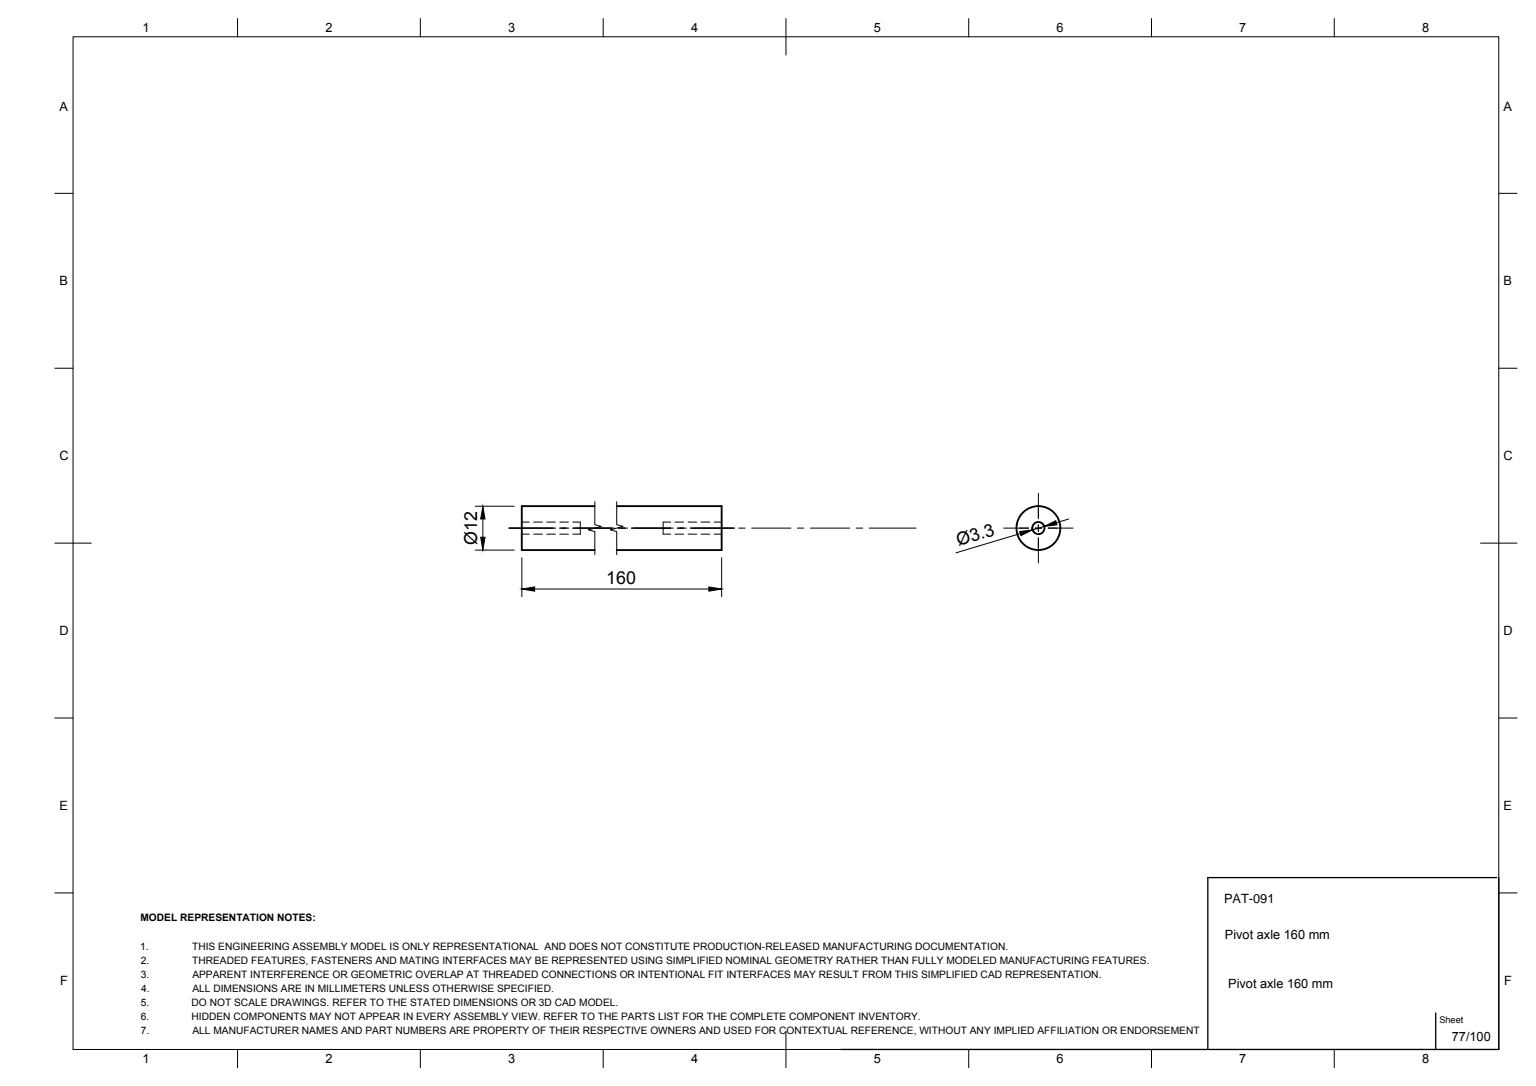
ISO-10303-21;
HEADER;
/* Generated by software containing ST-Developer
 * from STEP Tools, Inc. (www.steptools.com) 
 */

FILE_DESCRIPTION(
/* description */ ('PAT-091'),
/* implementation_level */ '2;1');

FILE_NAME(
/* name */ 'Pivot axle 160 mm.step',
/* time_stamp */ '2026-10-27T15:34:44-07:00',
/* author */ (''),
/* organization */ (''),
/* preprocessor_version */ 'ST-DEVELOPER v20.2',
/* originating_system */ 'Autodesk Translation Framework v15.17.0.0',
/* authorisation */ '');

FILE_SCHEMA (('AUTOMOTIVE_DESIGN { 1 0 10303 214 3 1 1 }'));
ENDSEC;

DATA;
#10=MECHANICAL_DESIGN_GEOMETRIC_PRESENTATION_REPRESENTATION('',(#1035),#25100);
#815=SHAPE_REPRESENTATION_RELATIONSHIP('SRR','None',#25581,#925);
#925=ADVANCED_BREP_SHAPE_REPRESENTATION('',(#1157),#25051);
#1035=STYLED_ITEM('',(#26191),#1157);
#1157=MANIFOLD_SOLID_BREP('Body1',#13314);
#1508=FACE_BOUND('',#3678,.T.);
#1509=FACE_BOUND('',#3680,.T.);
#1919=PLANE('',#15600);
#1920=PLANE('',#15604);
#1921=PLANE('',#15608);
#1922=PLANE('',#15609);
#2561=FACE_OUTER_BOUND('',#3672,.T.);
#2562=FACE_OUTER_BOUND('',#3673,.T.);
#2563=FACE_OUTER_BOUND('',#3674,.T.);
#2564=FACE_OUTER_BOUND('',#3675,.T.);
#2565=FACE_OUTER_BOUND('',#3676,.T.);
#2566=FACE_OUTER_BOUND('',#3677,.T.);
#2567=FACE_OUTER_BOUND('',#3679,.T.);
#3672=EDGE_LOOP('',(#10978,#10979,#10980,#10981));
#3673=EDGE_LOOP('',(#10982));
#3674=EDGE_LOOP('',(#10983,#10984,#10985,#10986));
#3675=EDGE_LOOP('',(#10987));
#3676=EDGE_LOOP('',(#10988,#10989,#10990,#10991));
#3677=EDGE_LOOP('',(#10992));
#3678=EDGE_LOOP('',(#10993));
#3679=EDGE_LOOP('',(#10994));
#3680=EDGE_LOOP('',(#10995));
#4683=LINE('',#23271,#5423);
#4684=LINE('',#23278,#5424);
#4685=LINE('',#23285,#5425);
#5423=VECTOR('',#19055,0.164999999999999);
#5424=VECTOR('',#19064,0.164999999999999);
#5425=VECTOR('',#19073,0.600000000000001);
#6044=CIRCLE('',#15598,0.164999999999999);
#6045=CIRCLE('',#15599,0.164999999999999);
#6046=CIRCLE('',#15602,0.164999999999999);
#6047=CIRCLE('',#15603,0.164999999999999);
#6048=CIRCLE('',#15606,0.600000000000001);
#6049=CIRCLE('',#15607,0.600000000000001);
#7049=VERTEX_POINT('',#23268);
#7050=VERTEX_POINT('',#23270);
#7051=VERTEX_POINT('',#23275);
#7052=VERTEX_POINT('',#23277);
#7053=VERTEX_POINT('',#23282);
#7054=VERTEX_POINT('',#23284);
#8424=EDGE_CURVE('',#7049,#7049,#6044,.T.);
#8425=EDGE_CURVE('',#7049,#7050,#4683,.T.);
#8426=EDGE_CURVE('',#7050,#7050,#6045,.T.);
#8427=EDGE_CURVE('',#7051,#7051,#6046,.T.);
#8428=EDGE_CURVE('',#7051,#7052,#4684,.T.);
#8429=EDGE_CURVE('',#7052,#7052,#6047,.T.);
#8430=EDGE_CURVE('',#7053,#7053,#6048,.T.);
#8431=EDGE_CURVE('',#7053,#7054,#4685,.T.);
#8432=EDGE_CURVE('',#7054,#7054,#6049,.T.);
#10978=ORIENTED_EDGE('',*,*,#8424,.F.);
#10979=ORIENTED_EDGE('',*,*,#8425,.T.);
#10980=ORIENTED_EDGE('',*,*,#8426,.F.);
#10981=ORIENTED_EDGE('',*,*,#8425,.F.);
#10982=ORIENTED_EDGE('',*,*,#8424,.T.);
#10983=ORIENTED_EDGE('',*,*,#8427,.F.);
#10984=ORIENTED_EDGE('',*,*,#8428,.T.);
#10985=ORIENTED_EDGE('',*,*,#8429,.T.);
#10986=ORIENTED_EDGE('',*,*,#8428,.F.);
#10987=ORIENTED_EDGE('',*,*,#8429,.F.);
#10988=ORIENTED_EDGE('',*,*,#8430,.F.);
#10989=ORIENTED_EDGE('',*,*,#8431,.T.);
#10990=ORIENTED_EDGE('',*,*,#8432,.T.);
#10991=ORIENTED_EDGE('',*,*,#8431,.F.);
#10992=ORIENTED_EDGE('',*,*,#8430,.T.);
#10993=ORIENTED_EDGE('',*,*,#8426,.T.);
#10994=ORIENTED_EDGE('',*,*,#8432,.F.);
#10995=ORIENTED_EDGE('',*,*,#8427,.T.);
#12285=CYLINDRICAL_SURFACE('',#15597,0.164999999999999);
#12286=CYLINDRICAL_SURFACE('',#15601,0.164999999999999);
#12287=CYLINDRICAL_SURFACE('',#15605,0.600000000000001);
#12928=ADVANCED_FACE('',(#2561),#12285,.F.);
#12929=ADVANCED_FACE('',(#2562),#1919,.T.);
#12930=ADVANCED_FACE('',(#2563),#12286,.F.);
#12931=ADVANCED_FACE('',(#2564),#1920,.F.);
#12932=ADVANCED_FACE('',(#2565),#12287,.T.);
#12933=ADVANCED_FACE('',(#2566,#1508),#1921,.T.);
#12934=ADVANCED_FACE('',(#2567,#1509),#1922,.F.);
#13314=CLOSED_SHELL('',(#12928,#12929,#12930,#12931,#12932,#12933,#12934));
#15596=AXIS2_PLACEMENT_3D('',#23266,#19049,#19050);
#15597=AXIS2_PLACEMENT_3D('',#23267,#19051,#19052);
#15598=AXIS2_PLACEMENT_3D('',#23269,#19053,#19054);
#15599=AXIS2_PLACEMENT_3D('',#23272,#19056,#19057);
#15600=AXIS2_PLACEMENT_3D('',#23273,#19058,#19059);
#15601=AXIS2_PLACEMENT_3D('',#23274,#19060,#19061);
#15602=AXIS2_PLACEMENT_3D('',#23276,#19062,#19063);
#15603=AXIS2_PLACEMENT_3D('',#23279,#19065,#19066);
#15604=AXIS2_PLACEMENT_3D('',#23280,#19067,#19068);
#15605=AXIS2_PLACEMENT_3D('',#23281,#19069,#19070);
#15606=AXIS2_PLACEMENT_3D('',#23283,#19071,#19072);
#15607=AXIS2_PLACEMENT_3D('',#23286,#19074,#19075);
#15608=AXIS2_PLACEMENT_3D('',#23287,#19076,#19077);
#15609=AXIS2_PLACEMENT_3D('',#23288,#19078,#19079);
#19049=DIRECTION('axis',(0.,0.,1.));
#19050=DIRECTION('refdir',(1.,0.,0.));
#19051=DIRECTION('center_axis',(0.,1.,0.));
#19052=DIRECTION('ref_axis',(1.,0.,0.));
#19053=DIRECTION('center_axis',(0.,1.,0.));
#19054=DIRECTION('ref_axis',(1.,0.,0.));
#19055=DIRECTION('',(0.,1.,0.));
#19056=DIRECTION('center_axis',(0.,-1.,0.));
#19057=DIRECTION('ref_axis',(1.,0.,0.));
#19058=DIRECTION('center_axis',(0.,1.,0.));
#19059=DIRECTION('ref_axis',(1.,0.,0.));
#19060=DIRECTION('center_axis',(0.,1.,0.));
#19061=DIRECTION('ref_axis',(1.,0.,0.));
#19062=DIRECTION('center_axis',(0.,1.,0.));
#19063=DIRECTION('ref_axis',(1.,0.,0.));
#19064=DIRECTION('',(0.,1.,0.));
#19065=DIRECTION('center_axis',(0.,1.,0.));
#19066=DIRECTION('ref_axis',(1.,0.,0.));
#19067=DIRECTION('center_axis',(0.,1.,0.));
#19068=DIRECTION('ref_axis',(1.,0.,0.));
#19069=DIRECTION('center_axis',(0.,1.,0.));
#19070=DIRECTION('ref_axis',(1.,0.,0.));
#19071=DIRECTION('center_axis',(0.,1.,0.));
#19072=DIRECTION('ref_axis',(1.,0.,0.));
#19073=DIRECTION('',(0.,-1.,0.));
#19074=DIRECTION('center_axis',(0.,1.,0.));
#19075=DIRECTION('ref_axis',(1.,0.,0.));
#19076=DIRECTION('center_axis',(0.,1.,0.));
#19077=DIRECTION('ref_axis',(1.,0.,0.));
#19078=DIRECTION('center_axis',(0.,1.,0.));
#19079=DIRECTION('ref_axis',(1.,0.,0.));
#23266=CARTESIAN_POINT('',(0.,0.,0.));
#23267=CARTESIAN_POINT('Origin',(19.3649167310371,6.9,8.));
#23268=CARTESIAN_POINT('',(19.1999167310371,6.9,8.));
#23269=CARTESIAN_POINT('Origin',(19.3649167310371,6.9,8.));
#23270=CARTESIAN_POINT('',(19.1999167310371,8.5,8.));
#23271=CARTESIAN_POINT('',(19.1999167310371,6.9,8.));
#23272=CARTESIAN_POINT('Origin',(19.3649167310371,8.5,8.));
#23273=CARTESIAN_POINT('Origin',(19.3649167310371,6.9,8.));
#23274=CARTESIAN_POINT('Origin',(19.3649167310371,-7.6,8.));
#23275=CARTESIAN_POINT('',(19.1999167310371,-7.5,8.));
#23276=CARTESIAN_POINT('Origin',(19.3649167310371,-7.5,8.));
#23277=CARTESIAN_POINT('',(19.1999167310371,-5.9,8.));
#23278=CARTESIAN_POINT('',(19.1999167310371,-7.6,8.));
#23279=CARTESIAN_POINT('Origin',(19.3649167310371,-5.9,8.));
#23280=CARTESIAN_POINT('Origin',(19.3649167310371,-5.9,8.));
#23281=CARTESIAN_POINT('Origin',(19.3649167310371,-7.5,8.));
#23282=CARTESIAN_POINT('',(18.7649167310371,8.5,8.));
#23283=CARTESIAN_POINT('Origin',(19.3649167310371,8.5,8.));
#23284=CARTESIAN_POINT('',(18.7649167310371,-7.5,8.));
#23285=CARTESIAN_POINT('',(18.7649167310371,-7.5,8.));
#23286=CARTESIAN_POINT('Origin',(19.3649167310371,-7.5,8.));
#23287=CARTESIAN_POINT('Origin',(19.3649167310371,8.5,8.));
#23288=CARTESIAN_POINT('Origin',(19.3649167310371,-7.5,8.));
#24930=UNCERTAINTY_MEASURE_WITH_UNIT(LENGTH_MEASURE(0.001),#25101,
'DISTANCE_ACCURACY_VALUE',
'Maximum model space distance between geometric entities at asserted c
onnectivities');
#24979=UNCERTAINTY_MEASURE_WITH_UNIT(LENGTH_MEASURE(0.001),#25101,
'DISTANCE_ACCURACY_VALUE',
'Maximum model space distance between geometric entities at asserted c
onnectivities');
#25051=(
GEOMETRIC_REPRESENTATION_CONTEXT(3)
GLOBAL_UNCERTAINTY_ASSIGNED_CONTEXT((#24930))
GLOBAL_UNIT_ASSIGNED_CONTEXT((#25101,#25103,#25104))
REPRESENTATION_CONTEXT('','3D')
);
#25100=(
GEOMETRIC_REPRESENTATION_CONTEXT(3)
GLOBAL_UNCERTAINTY_ASSIGNED_CONTEXT((#24979))
GLOBAL_UNIT_ASSIGNED_CONTEXT((#25101,#25103,#25104))
REPRESENTATION_CONTEXT('','3D')
);
#25101=(
LENGTH_UNIT()
NAMED_UNIT(*)
SI_UNIT(.CENTI.,.METRE.)
);
#25103=(
NAMED_UNIT(*)
PLANE_ANGLE_UNIT()
SI_UNIT($,.RADIAN.)
);
#25104=(
NAMED_UNIT(*)
SI_UNIT($,.STERADIAN.)
SOLID_ANGLE_UNIT()
);
#25176=SHAPE_DEFINITION_REPRESENTATION(#25298,#25581);
#25298=PRODUCT_DEFINITION_SHAPE('',$,#25702);
#25581=SHAPE_REPRESENTATION('',(#15596),#25051);
#25630=PRODUCT_DEFINITION_CONTEXT('part definition',#25992,'design');
#25702=PRODUCT_DEFINITION('Pivot axle 160 mm','Pivot axle 160 mm',#25822,
#25630);
#25822=PRODUCT_DEFINITION_FORMATION('',$,#26065);
#25992=APPLICATION_CONTEXT(
'Core Data for Automotive Mechanical Design Process');
#25993=PRODUCT_CONTEXT('part definition',#25992,'mechanical');
#26065=PRODUCT('Pivot axle 160 mm','Pivot axle 160 mm',
'Pivot axle 160 mm',(#25993));
#26185=COLOUR_RGB('Grey',0.48,0.52,0.57);
#26186=FILL_AREA_STYLE_COLOUR('',#26185);
#26187=FILL_AREA_STYLE('',(#26186));
#26188=SURFACE_STYLE_FILL_AREA(#26187);
#26189=SURFACE_SIDE_STYLE('',(#26188));
#26190=SURFACE_STYLE_USAGE(.BOTH.,#26189);
#26191=PRESENTATION_STYLE_ASSIGNMENT((#26190));
ENDSEC;
END-ISO-10303-21;
